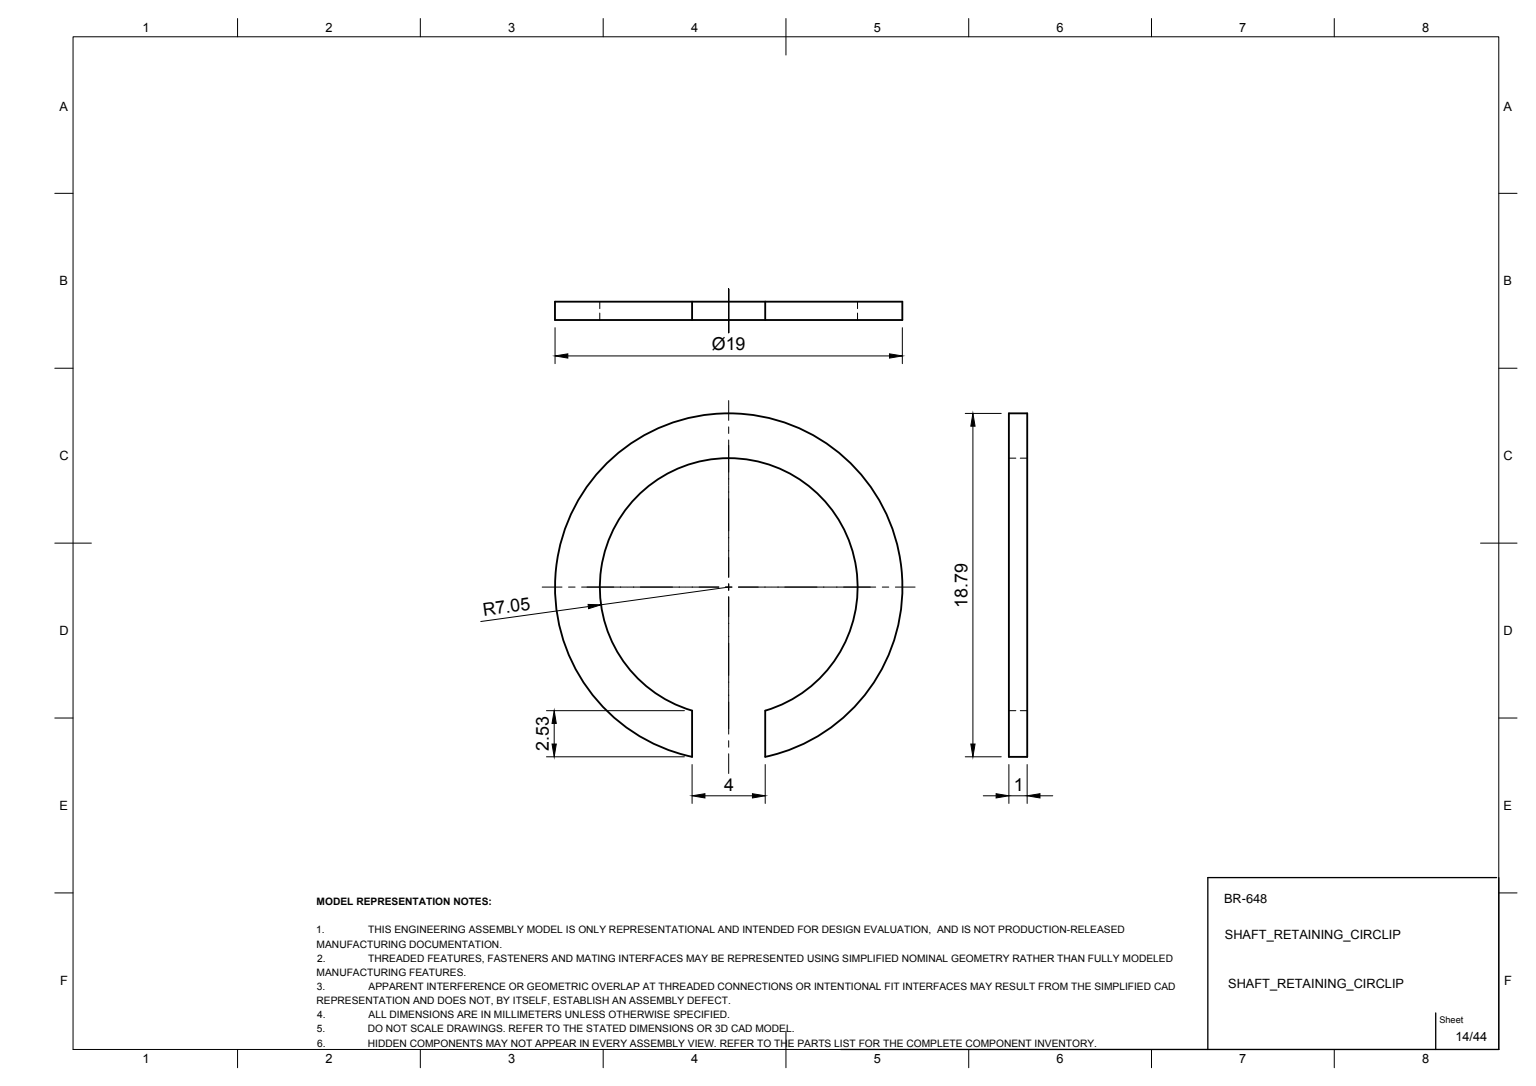
ISO-10303-21;
HEADER;
FILE_DESCRIPTION((''),'2;1');
FILE_NAME('SHAFT_RETAINING_CIRCLIP.step','2026-10-01T22:05:39-07:00',(''),(''),'','','');
FILE_SCHEMA (('AUTOMOTIVE_DESIGN { 1 0 10303 214 3 1 1 }'));
ENDSEC;
DATA;
#10=MECHANICAL_DESIGN_GEOMETRIC_PRESENTATION_REPRESENTATION('',(#614),#24628);
#530=SHAPE_REPRESENTATION_RELATIONSHIP('SRR','None',#24802,#572) ;
#572=ADVANCED_BREP_SHAPE_REPRESENTATION('',(#654),#24592) ;
#614=STYLED_ITEM('',(#25030),#654) ;
#654=MANIFOLD_SOLID_BREP('SHAFT_RETAINING_CIRCLIP',#13125) ;
#1152=LINE('',#20686,#1988) ;
#1153=LINE('',#20688,#1989) ;
#1154=LINE('',#20690,#1990) ;
#1155=LINE('',#20691,#1991) ;
#1156=LINE('',#20695,#1992) ;
#1157=LINE('',#20697,#1993) ;
#1158=LINE('',#20699,#1994) ;
#1159=LINE('',#20700,#1995) ;
#1988=VECTOR('',#16449,1.) ;
#1989=VECTOR('',#16450,1.) ;
#1990=VECTOR('',#16451,1.) ;
#1991=VECTOR('',#16452,1.) ;
#1992=VECTOR('',#16455,1.) ;
#1993=VECTOR('',#16456,1.) ;
#1994=VECTOR('',#16457,1.) ;
#1995=VECTOR('',#16458,1.) ;
#2788=CYLINDRICAL_SURFACE('',#14110,0.705) ;
#2789=CYLINDRICAL_SURFACE('',#14112,0.95) ;
#3144=FACE_OUTER_BOUND('',#4074,.T.) ;
#3145=FACE_OUTER_BOUND('',#4075,.T.) ;
#3146=FACE_OUTER_BOUND('',#4076,.T.) ;
#3147=FACE_OUTER_BOUND('',#4077,.T.) ;
#3148=FACE_OUTER_BOUND('',#4078,.T.) ;
#3149=FACE_OUTER_BOUND('',#4079,.T.) ;
#4074=EDGE_LOOP('',(#9297,#9298,#9299,#9300)) ;
#4075=EDGE_LOOP('',(#9301,#9302,#9303,#9304)) ;
#4076=EDGE_LOOP('',(#9305,#9306,#9307,#9308)) ;
#4077=EDGE_LOOP('',(#9309,#9310,#9311,#9312)) ;
#4078=EDGE_LOOP('',(#9313,#9314,#9315,#9316)) ;
#4079=EDGE_LOOP('',(#9317,#9318,#9319,#9320)) ;
#5000=CIRCLE('',#14108,0.95) ;
#5001=CIRCLE('',#14109,0.705) ;
#5002=CIRCLE('',#14111,0.705) ;
#5003=CIRCLE('',#14113,0.95) ;
#5807=VERTEX_POINT('',#20684) ;
#5808=VERTEX_POINT('',#20685) ;
#5809=VERTEX_POINT('',#20687) ;
#5810=VERTEX_POINT('',#20689) ;
#5811=VERTEX_POINT('',#20693) ;
#5812=VERTEX_POINT('',#20694) ;
#5813=VERTEX_POINT('',#20696) ;
#5814=VERTEX_POINT('',#20698) ;
#7138=EDGE_CURVE('',#5807,#5808,#1152,.T.) ;
#7139=EDGE_CURVE('',#5809,#5807,#1153,.T.) ;
#7140=EDGE_CURVE('',#5810,#5809,#1154,.T.) ;
#7141=EDGE_CURVE('',#5808,#5810,#1155,.T.) ;
#7142=EDGE_CURVE('',#5811,#5812,#1156,.T.) ;
#7143=EDGE_CURVE('',#5813,#5811,#1157,.T.) ;
#7144=EDGE_CURVE('',#5814,#5813,#1158,.T.) ;
#7145=EDGE_CURVE('',#5812,#5814,#1159,.T.) ;
#7146=EDGE_CURVE('',#5807,#5812,#5000,.T.) ;
#7147=EDGE_CURVE('',#5814,#5809,#5001,.T.) ;
#7148=EDGE_CURVE('',#5810,#5813,#5002,.T.) ;
#7149=EDGE_CURVE('',#5811,#5808,#5003,.T.) ;
#9297=ORIENTED_EDGE('',*,*,#7138,.F.) ;
#9298=ORIENTED_EDGE('',*,*,#7139,.F.) ;
#9299=ORIENTED_EDGE('',*,*,#7140,.F.) ;
#9300=ORIENTED_EDGE('',*,*,#7141,.F.) ;
#9301=ORIENTED_EDGE('',*,*,#7142,.F.) ;
#9302=ORIENTED_EDGE('',*,*,#7143,.F.) ;
#9303=ORIENTED_EDGE('',*,*,#7144,.F.) ;
#9304=ORIENTED_EDGE('',*,*,#7145,.F.) ;
#9305=ORIENTED_EDGE('',*,*,#7139,.T.) ;
#9306=ORIENTED_EDGE('',*,*,#7146,.T.) ;
#9307=ORIENTED_EDGE('',*,*,#7145,.T.) ;
#9308=ORIENTED_EDGE('',*,*,#7147,.T.) ;
#9309=ORIENTED_EDGE('',*,*,#7140,.T.) ;
#9310=ORIENTED_EDGE('',*,*,#7147,.F.) ;
#9311=ORIENTED_EDGE('',*,*,#7144,.T.) ;
#9312=ORIENTED_EDGE('',*,*,#7148,.F.) ;
#9313=ORIENTED_EDGE('',*,*,#7138,.T.) ;
#9314=ORIENTED_EDGE('',*,*,#7149,.F.) ;
#9315=ORIENTED_EDGE('',*,*,#7142,.T.) ;
#9316=ORIENTED_EDGE('',*,*,#7146,.F.) ;
#9317=ORIENTED_EDGE('',*,*,#7141,.T.) ;
#9318=ORIENTED_EDGE('',*,*,#7148,.T.) ;
#9319=ORIENTED_EDGE('',*,*,#7143,.T.) ;
#9320=ORIENTED_EDGE('',*,*,#7149,.T.) ;
#12072=PLANE('',#14105) ;
#12073=PLANE('',#14106) ;
#12074=PLANE('',#14107) ;
#12075=PLANE('',#14114) ;
#12539=ADVANCED_FACE('',(#3144),#12072,.T.) ;
#12540=ADVANCED_FACE('',(#3145),#12073,.T.) ;
#12541=ADVANCED_FACE('',(#3146),#12074,.T.) ;
#12542=ADVANCED_FACE('',(#3147),#2788,.F.) ;
#12543=ADVANCED_FACE('',(#3148),#2789,.T.) ;
#12544=ADVANCED_FACE('',(#3149),#12075,.T.) ;
#13125=CLOSED_SHELL('',(#12539,#12540,#12541,#12542,#12543,#12544)) ;
#14104=AXIS2_PLACEMENT_3D('',#20682,#16445,#16446) ;
#14105=AXIS2_PLACEMENT_3D('',#20683,#16447,#16448) ;
#14106=AXIS2_PLACEMENT_3D('',#20692,#16453,#16454) ;
#14107=AXIS2_PLACEMENT_3D('',#20701,#16459,#16460) ;
#14108=AXIS2_PLACEMENT_3D('',#20702,#16461,#16462) ;
#14109=AXIS2_PLACEMENT_3D('',#20703,#16463,#16464) ;
#14110=AXIS2_PLACEMENT_3D('',#20704,#16465,#16466) ;
#14111=AXIS2_PLACEMENT_3D('',#20705,#16467,#16468) ;
#14112=AXIS2_PLACEMENT_3D('',#20706,#16469,#16470) ;
#14113=AXIS2_PLACEMENT_3D('',#20707,#16471,#16472) ;
#14114=AXIS2_PLACEMENT_3D('',#20708,#16473,#16474) ;
#16445=DIRECTION('axis',(0.,0.,1.)) ;
#16446=DIRECTION('refdir',(1.,0.,0.)) ;
#16447=DIRECTION('center_axis',(1.,0.,0.)) ;
#16448=DIRECTION('ref_axis',(0.,0.,-1.)) ;
#16449=DIRECTION('',(0.,-1.,0.)) ;
#16450=DIRECTION('',(0.,0.,-1.)) ;
#16451=DIRECTION('',(0.,1.,0.)) ;
#16452=DIRECTION('',(0.,0.,1.)) ;
#16453=DIRECTION('center_axis',(-1.,0.,0.)) ;
#16454=DIRECTION('ref_axis',(0.,0.,1.)) ;
#16455=DIRECTION('',(0.,1.,0.)) ;
#16456=DIRECTION('',(0.,0.,-1.)) ;
#16457=DIRECTION('',(0.,-1.,0.)) ;
#16458=DIRECTION('',(0.,0.,1.)) ;
#16459=DIRECTION('center_axis',(0.,1.,0.)) ;
#16460=DIRECTION('ref_axis',(1.,0.,0.)) ;
#16461=DIRECTION('center_axis',(0.,1.,0.)) ;
#16462=DIRECTION('ref_axis',(1.,0.,0.)) ;
#16463=DIRECTION('center_axis',(0.,-1.,0.)) ;
#16464=DIRECTION('ref_axis',(1.,0.,0.)) ;
#16465=DIRECTION('center_axis',(0.,1.,0.)) ;
#16466=DIRECTION('ref_axis',(-1.83697019872103E-16,0.,1.)) ;
#16467=DIRECTION('center_axis',(0.,1.,0.)) ;
#16468=DIRECTION('ref_axis',(1.,0.,0.)) ;
#16469=DIRECTION('center_axis',(0.,1.,0.)) ;
#16470=DIRECTION('ref_axis',(-1.83697019872103E-16,0.,1.)) ;
#16471=DIRECTION('center_axis',(0.,-1.,0.)) ;
#16472=DIRECTION('ref_axis',(1.,0.,0.)) ;
#16473=DIRECTION('center_axis',(0.,-1.,0.)) ;
#16474=DIRECTION('ref_axis',(-1.,0.,0.)) ;
#20682=CARTESIAN_POINT('',(0.,0.,0.)) ;
#20683=CARTESIAN_POINT('Origin',(-0.2,-5.25,-0.8)) ;
#20684=CARTESIAN_POINT('',(-0.2,-5.2,-0.928708781050335)) ;
#20685=CARTESIAN_POINT('',(-0.2,-5.3,-0.928708781050335)) ;
#20686=CARTESIAN_POINT('',(-0.2,-5.25,-0.928708781050335)) ;
#20687=CARTESIAN_POINT('',(-0.2,-5.2,-0.676036241632059)) ;
#20688=CARTESIAN_POINT('',(-0.2,-5.2,-0.4)) ;
#20689=CARTESIAN_POINT('',(-0.2,-5.3,-0.676036241632059)) ;
#20690=CARTESIAN_POINT('',(-0.2,-5.25,-0.676036241632059)) ;
#20691=CARTESIAN_POINT('',(-0.2,-5.3,-0.4)) ;
#20692=CARTESIAN_POINT('Origin',(0.2,-5.25,-0.8)) ;
#20693=CARTESIAN_POINT('',(0.2,-5.3,-0.928708781050335)) ;
#20694=CARTESIAN_POINT('',(0.2,-5.2,-0.928708781050335)) ;
#20695=CARTESIAN_POINT('',(0.2,-5.25,-0.928708781050335)) ;
#20696=CARTESIAN_POINT('',(0.2,-5.3,-0.676036241632059)) ;
#20697=CARTESIAN_POINT('',(0.2,-5.3,-0.4)) ;
#20698=CARTESIAN_POINT('',(0.2,-5.2,-0.676036241632059)) ;
#20699=CARTESIAN_POINT('',(0.2,-5.25,-0.676036241632059)) ;
#20700=CARTESIAN_POINT('',(0.2,-5.2,-0.4)) ;
#20701=CARTESIAN_POINT('Origin',(0.,-5.2,0.)) ;
#20702=CARTESIAN_POINT('Origin',(0.,-5.2,0.)) ;
#20703=CARTESIAN_POINT('Origin',(0.,-5.2,0.)) ;
#20704=CARTESIAN_POINT('Origin',(0.,-5.25,0.)) ;
#20705=CARTESIAN_POINT('Origin',(0.,-5.3,0.)) ;
#20706=CARTESIAN_POINT('Origin',(0.,-5.25,0.)) ;
#20707=CARTESIAN_POINT('Origin',(0.,-5.3,0.)) ;
#20708=CARTESIAN_POINT('Origin',(0.,-5.3,0.)) ;
#24544=UNCERTAINTY_MEASURE_WITH_UNIT(LENGTH_MEASURE(0.001),#24629,
'DISTANCE_ACCURACY_VALUE',
'Maximum model space distance between geometric entities at asserted c
onnectivities') ;
#24580=UNCERTAINTY_MEASURE_WITH_UNIT(LENGTH_MEASURE(0.001),#24629,
'DISTANCE_ACCURACY_VALUE',
'Maximum model space distance between geometric entities at asserted c
onnectivities') ;
#24592=(
GEOMETRIC_REPRESENTATION_CONTEXT(3)
GLOBAL_UNCERTAINTY_ASSIGNED_CONTEXT((#24544))
GLOBAL_UNIT_ASSIGNED_CONTEXT((#24629,#24631,#24632))
REPRESENTATION_CONTEXT('','3D')
) ;
#24628=(
GEOMETRIC_REPRESENTATION_CONTEXT(3)
GLOBAL_UNCERTAINTY_ASSIGNED_CONTEXT((#24580))
GLOBAL_UNIT_ASSIGNED_CONTEXT((#24629,#24631,#24632))
REPRESENTATION_CONTEXT('','3D')
) ;
#24629=(
LENGTH_UNIT()
NAMED_UNIT(*)
SI_UNIT(.CENTI.,.METRE.)
) ;
#24631=(
NAMED_UNIT(*)
PLANE_ANGLE_UNIT()
SI_UNIT($,.RADIAN.)
) ;
#24632=(
NAMED_UNIT(*)
SI_UNIT($,.STERADIAN.)
SOLID_ANGLE_UNIT()
) ;
#24644=SHAPE_DEFINITION_REPRESENTATION(#24691,#24802) ;
#24691=PRODUCT_DEFINITION_SHAPE('',$,#24850) ;
#24802=SHAPE_REPRESENTATION('',(#14104),#24592) ;
#24838=PRODUCT_DEFINITION_CONTEXT('part definition',#24981,'design') ;
#24850=PRODUCT_DEFINITION('SHAFT_RETAINING_CIRCLIP',
'SHAFT_RETAINING_CIRCLIP',#24897,#24838) ;
#24897=PRODUCT_DEFINITION_FORMATION('',$,#24994) ;
#24981=APPLICATION_CONTEXT(
'Core Data for Automotive Mechanical Design Process') ;
#24982=PRODUCT_CONTEXT('part definition',#24981,'mechanical') ;
#24994=PRODUCT('SHAFT_RETAINING_CIRCLIP','SHAFT_RETAINING_CIRCLIP',$,(#24982)) ;
#25030=PRESENTATION_STYLE_ASSIGNMENT((#25040)) ;
#25040=SURFACE_STYLE_USAGE(.BOTH.,#25050) ;
#25050=SURFACE_SIDE_STYLE('',(#25060)) ;
#25060=SURFACE_STYLE_FILL_AREA(#25070) ;
#25070=FILL_AREA_STYLE('Steel - Satin',(#25080)) ;
#25080=FILL_AREA_STYLE_COLOUR('Steel - Satin',#25090) ;
#25090=COLOUR_RGB('Steel - Satin', 0.66274510, 0.83137255, 0.94901961) ;
ENDSEC;
END-ISO-10303-21;
